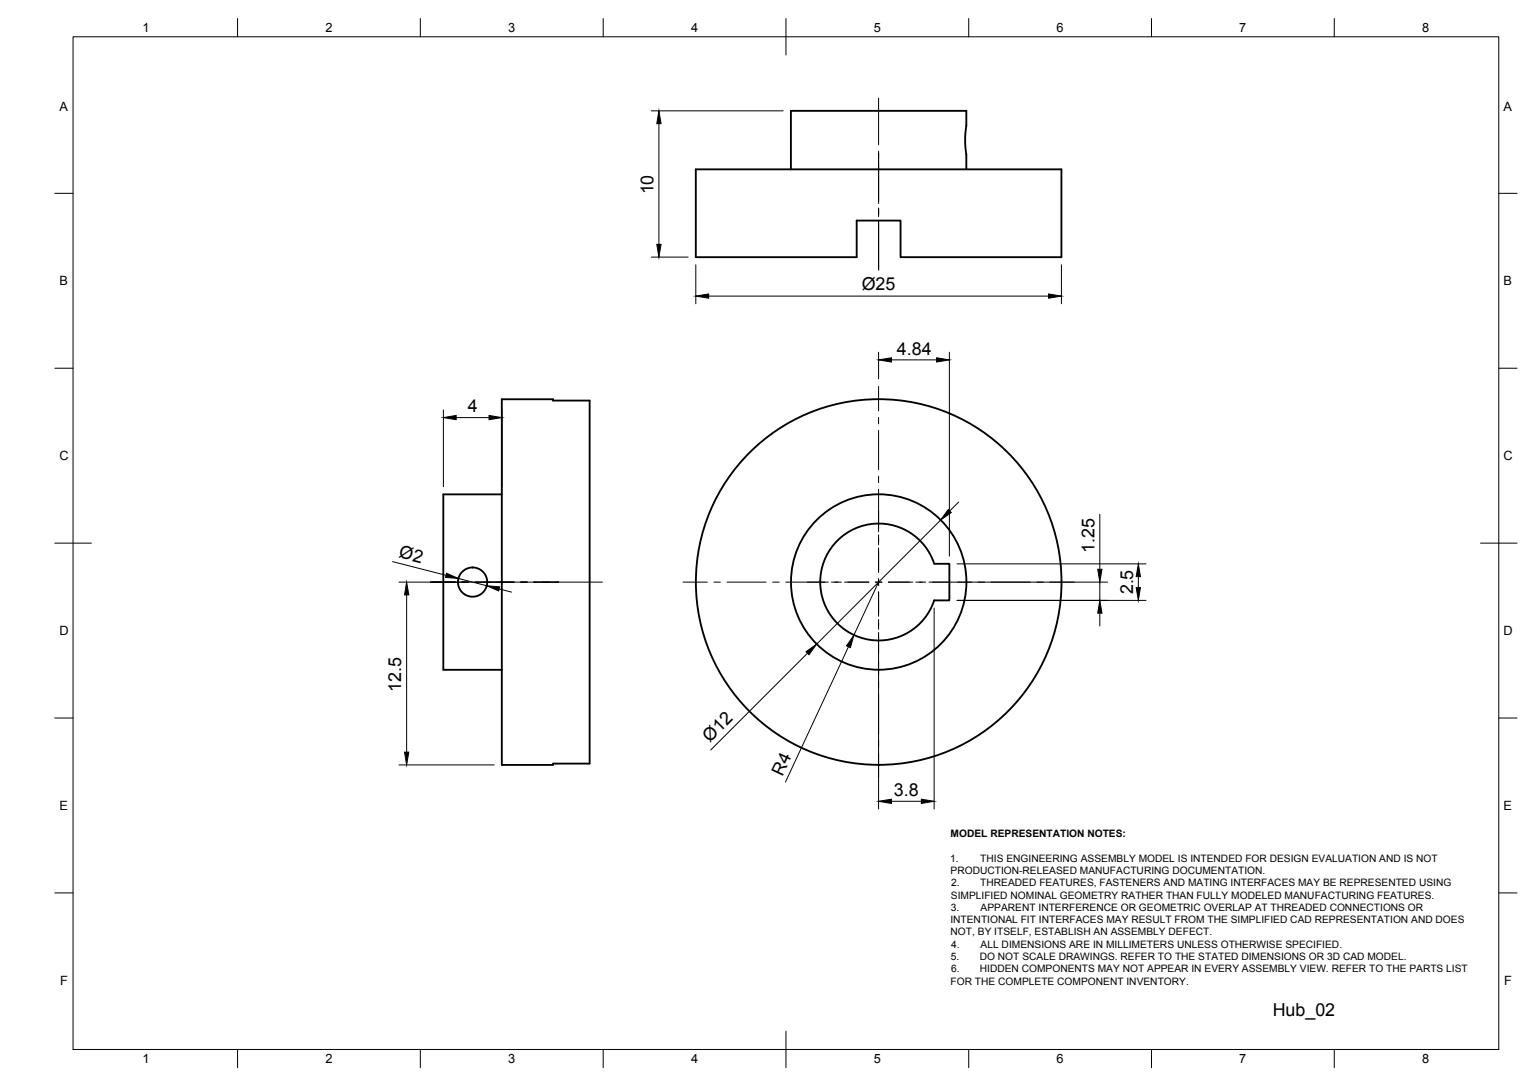
ISO-10303-21;
HEADER;
/* Generated by software containing ST-Developer
 * from STEP Tools, Inc. (www.steptools.com) 
 */

FILE_DESCRIPTION(
/* description */ (''),
/* implementation_level */ '2;1');

FILE_NAME(
/* name */ 'Hub_02.step',
/* time_stamp */ '2026-10-05T22:24:12-07:00',
/* author */ (''),
/* organization */ (''),
/* preprocessor_version */ 'ST-DEVELOPER v20.2',
/* originating_system */ 'Autodesk Translation Framework v15.15.0.0',
/* authorisation */ '');

FILE_SCHEMA (('AUTOMOTIVE_DESIGN { 1 0 10303 214 3 1 1 }'));
ENDSEC;

DATA;
#10=MECHANICAL_DESIGN_GEOMETRIC_PRESENTATION_REPRESENTATION('',(#55),#2116);
#41=SHAPE_REPRESENTATION_RELATIONSHIP('SRR','None',#2147,#48);
#48=ADVANCED_BREP_SHAPE_REPRESENTATION('',(#62),#2111);
#55=STYLED_ITEM('',(#2191),#62);
#62=MANIFOLD_SOLID_BREP('Body1',#1149);
#71=FACE_BOUND('',#230,.T.);
#72=FACE_BOUND('',#234,.T.);
#73=FACE_BOUND('',#237,.T.);
#74=FACE_BOUND('',#239,.T.);
#96=PLANE('',#1285);
#97=PLANE('',#1286);
#98=PLANE('',#1287);
#99=PLANE('',#1288);
#100=PLANE('',#1295);
#101=PLANE('',#1297);
#102=PLANE('',#1298);
#103=PLANE('',#1299);
#104=PLANE('',#1303);
#105=PLANE('',#1305);
#106=PLANE('',#1308);
#157=FACE_OUTER_BOUND('',#228,.T.);
#158=FACE_OUTER_BOUND('',#229,.T.);
#159=FACE_OUTER_BOUND('',#231,.T.);
#160=FACE_OUTER_BOUND('',#232,.T.);
#161=FACE_OUTER_BOUND('',#233,.T.);
#162=FACE_OUTER_BOUND('',#235,.T.);
#163=FACE_OUTER_BOUND('',#236,.T.);
#164=FACE_OUTER_BOUND('',#238,.T.);
#165=FACE_OUTER_BOUND('',#240,.T.);
#166=FACE_OUTER_BOUND('',#241,.T.);
#167=FACE_OUTER_BOUND('',#242,.T.);
#168=FACE_OUTER_BOUND('',#243,.T.);
#169=FACE_OUTER_BOUND('',#244,.T.);
#170=FACE_OUTER_BOUND('',#245,.T.);
#171=FACE_OUTER_BOUND('',#246,.T.);
#228=EDGE_LOOP('',(#893,#894,#895,#896,#897));
#229=EDGE_LOOP('',(#898,#899,#900,#901));
#230=EDGE_LOOP('',(#902));
#231=EDGE_LOOP('',(#903,#904,#905,#906));
#232=EDGE_LOOP('',(#907,#908,#909,#910));
#233=EDGE_LOOP('',(#911));
#234=EDGE_LOOP('',(#912,#913,#914,#915));
#235=EDGE_LOOP('',(#916,#917,#918,#919));
#236=EDGE_LOOP('',(#920,#921,#922,#923));
#237=EDGE_LOOP('',(#924,#925));
#238=EDGE_LOOP('',(#926));
#239=EDGE_LOOP('',(#927));
#240=EDGE_LOOP('',(#928,#929,#930,#931));
#241=EDGE_LOOP('',(#932,#933,#934,#935));
#242=EDGE_LOOP('',(#936,#937,#938,#939,#940));
#243=EDGE_LOOP('',(#941,#942));
#244=EDGE_LOOP('',(#943,#944));
#245=EDGE_LOOP('',(#945,#946,#947,#948,#949,#950,#951,#952,#953,#954,#955,
#956));
#246=EDGE_LOOP('',(#957,#958,#959,#960));
#274=B_SPLINE_CURVE_WITH_KNOTS('',3,(#1872,#1873,#1874,#1875,#1876,#1877,
#1878,#1879,#1880,#1881,#1882,#1883,#1884,#1885,#1886,#1887,#1888,#1889),
 .UNSPECIFIED.,.F.,.F.,(4,2,2,2,2,2,2,2,4),(0.,0.0377449625945587,0.0754899251891175,
0.113233879657538,0.150977834125959,0.18872178859438,0.226465743062801,
0.264210705657359,0.301955668251918),.UNSPECIFIED.);
#275=B_SPLINE_CURVE_WITH_KNOTS('',3,(#1890,#1891,#1892,#1893,#1894,#1895,
#1896,#1897,#1898,#1899,#1900,#1901,#1902,#1903,#1904,#1905,#1906,#1907),
 .UNSPECIFIED.,.F.,.F.,(4,2,2,2,2,2,2,2,4),(0.301955668251918,0.339700630846477,
0.377445593441036,0.415189547909457,0.452933502377877,0.490677456846298,
0.528421411314719,0.566166373909278,0.603911336503836),.UNSPECIFIED.);
#314=LINE('',#1870,#419);
#315=LINE('',#1911,#420);
#316=LINE('',#1913,#421);
#317=LINE('',#1915,#422);
#318=LINE('',#1916,#423);
#319=LINE('',#1919,#424);
#320=LINE('',#1921,#425);
#321=LINE('',#1922,#426);
#322=LINE('',#1925,#427);
#323=LINE('',#1927,#428);
#324=LINE('',#1928,#429);
#325=LINE('',#1937,#430);
#326=LINE('',#1945,#431);
#327=LINE('',#1947,#432);
#328=LINE('',#1949,#433);
#329=LINE('',#1950,#434);
#330=LINE('',#1954,#435);
#331=LINE('',#1956,#436);
#332=LINE('',#1958,#437);
#333=LINE('',#1959,#438);
#334=LINE('',#1970,#439);
#419=VECTOR('',#1498,0.999999999999999);
#420=VECTOR('',#1501,10.);
#421=VECTOR('',#1502,10.);
#422=VECTOR('',#1503,10.);
#423=VECTOR('',#1504,10.);
#424=VECTOR('',#1507,10.);
#425=VECTOR('',#1508,10.);
#426=VECTOR('',#1509,10.);
#427=VECTOR('',#1512,10.);
#428=VECTOR('',#1513,10.);
#429=VECTOR('',#1514,10.);
#430=VECTOR('',#1527,6.);
#431=VECTOR('',#1536,10.);
#432=VECTOR('',#1537,10.);
#433=VECTOR('',#1538,10.);
#434=VECTOR('',#1539,10.);
#435=VECTOR('',#1542,10.);
#436=VECTOR('',#1543,10.);
#437=VECTOR('',#1544,10.);
#438=VECTOR('',#1545,10.);
#439=VECTOR('',#1564,12.5);
#507=CIRCLE('',#1284,0.999999999999999);
#508=CIRCLE('',#1289,6.);
#509=CIRCLE('',#1290,4.);
#510=CIRCLE('',#1292,4.);
#511=CIRCLE('',#1294,6.);
#512=CIRCLE('',#1296,12.5);
#513=CIRCLE('',#1300,12.5);
#514=CIRCLE('',#1301,12.5);
#515=CIRCLE('',#1302,12.5);
#516=CIRCLE('',#1304,12.5);
#517=CIRCLE('',#1306,12.5);
#566=VERTEX_POINT('',#1867);
#567=VERTEX_POINT('',#1869);
#568=VERTEX_POINT('',#1871);
#569=VERTEX_POINT('',#1909);
#570=VERTEX_POINT('',#1910);
#571=VERTEX_POINT('',#1912);
#572=VERTEX_POINT('',#1914);
#573=VERTEX_POINT('',#1918);
#574=VERTEX_POINT('',#1920);
#575=VERTEX_POINT('',#1924);
#576=VERTEX_POINT('',#1926);
#577=VERTEX_POINT('',#1930);
#578=VERTEX_POINT('',#1936);
#579=VERTEX_POINT('',#1940);
#580=VERTEX_POINT('',#1943);
#581=VERTEX_POINT('',#1944);
#582=VERTEX_POINT('',#1946);
#583=VERTEX_POINT('',#1948);
#584=VERTEX_POINT('',#1952);
#585=VERTEX_POINT('',#1953);
#586=VERTEX_POINT('',#1955);
#587=VERTEX_POINT('',#1957);
#588=VERTEX_POINT('',#1962);
#685=EDGE_CURVE('',#566,#566,#507,.T.);
#686=EDGE_CURVE('',#566,#567,#314,.T.);
#687=EDGE_CURVE('',#568,#567,#274,.T.);
#688=EDGE_CURVE('',#567,#568,#275,.T.);
#689=EDGE_CURVE('',#569,#570,#315,.T.);
#690=EDGE_CURVE('',#571,#569,#316,.T.);
#691=EDGE_CURVE('',#572,#571,#317,.T.);
#692=EDGE_CURVE('',#572,#570,#318,.T.);
#693=EDGE_CURVE('',#570,#573,#319,.T.);
#694=EDGE_CURVE('',#572,#574,#320,.T.);
#695=EDGE_CURVE('',#573,#574,#321,.T.);
#696=EDGE_CURVE('',#575,#569,#322,.T.);
#697=EDGE_CURVE('',#576,#575,#323,.T.);
#698=EDGE_CURVE('',#571,#576,#324,.T.);
#699=EDGE_CURVE('',#577,#577,#508,.T.);
#700=EDGE_CURVE('',#573,#575,#509,.T.);
#701=EDGE_CURVE('',#576,#574,#510,.T.);
#702=EDGE_CURVE('',#577,#578,#325,.T.);
#703=EDGE_CURVE('',#578,#578,#511,.T.);
#704=EDGE_CURVE('',#579,#579,#512,.T.);
#705=EDGE_CURVE('',#580,#581,#326,.T.);
#706=EDGE_CURVE('',#582,#580,#327,.T.);
#707=EDGE_CURVE('',#582,#583,#328,.T.);
#708=EDGE_CURVE('',#581,#583,#329,.T.);
#709=EDGE_CURVE('',#584,#585,#330,.T.);
#710=EDGE_CURVE('',#586,#584,#331,.T.);
#711=EDGE_CURVE('',#586,#587,#332,.T.);
#712=EDGE_CURVE('',#585,#587,#333,.T.);
#713=EDGE_CURVE('',#583,#586,#513,.T.);
#714=EDGE_CURVE('',#588,#582,#514,.T.);
#715=EDGE_CURVE('',#587,#588,#515,.T.);
#716=EDGE_CURVE('',#584,#585,#516,.T.);
#717=EDGE_CURVE('',#580,#581,#517,.T.);
#718=EDGE_CURVE('',#579,#588,#334,.T.);
#893=ORIENTED_EDGE('',*,*,#685,.F.);
#894=ORIENTED_EDGE('',*,*,#686,.T.);
#895=ORIENTED_EDGE('',*,*,#687,.F.);
#896=ORIENTED_EDGE('',*,*,#688,.F.);
#897=ORIENTED_EDGE('',*,*,#686,.F.);
#898=ORIENTED_EDGE('',*,*,#689,.F.);
#899=ORIENTED_EDGE('',*,*,#690,.F.);
#900=ORIENTED_EDGE('',*,*,#691,.F.);
#901=ORIENTED_EDGE('',*,*,#692,.T.);
#902=ORIENTED_EDGE('',*,*,#685,.T.);
#903=ORIENTED_EDGE('',*,*,#693,.F.);
#904=ORIENTED_EDGE('',*,*,#692,.F.);
#905=ORIENTED_EDGE('',*,*,#694,.T.);
#906=ORIENTED_EDGE('',*,*,#695,.F.);
#907=ORIENTED_EDGE('',*,*,#696,.F.);
#908=ORIENTED_EDGE('',*,*,#697,.F.);
#909=ORIENTED_EDGE('',*,*,#698,.F.);
#910=ORIENTED_EDGE('',*,*,#690,.T.);
#911=ORIENTED_EDGE('',*,*,#699,.T.);
#912=ORIENTED_EDGE('',*,*,#696,.T.);
#913=ORIENTED_EDGE('',*,*,#689,.T.);
#914=ORIENTED_EDGE('',*,*,#693,.T.);
#915=ORIENTED_EDGE('',*,*,#700,.T.);
#916=ORIENTED_EDGE('',*,*,#697,.T.);
#917=ORIENTED_EDGE('',*,*,#700,.F.);
#918=ORIENTED_EDGE('',*,*,#695,.T.);
#919=ORIENTED_EDGE('',*,*,#701,.F.);
#920=ORIENTED_EDGE('',*,*,#699,.F.);
#921=ORIENTED_EDGE('',*,*,#702,.T.);
#922=ORIENTED_EDGE('',*,*,#703,.F.);
#923=ORIENTED_EDGE('',*,*,#702,.F.);
#924=ORIENTED_EDGE('',*,*,#687,.T.);
#925=ORIENTED_EDGE('',*,*,#688,.T.);
#926=ORIENTED_EDGE('',*,*,#704,.T.);
#927=ORIENTED_EDGE('',*,*,#703,.T.);
#928=ORIENTED_EDGE('',*,*,#705,.F.);
#929=ORIENTED_EDGE('',*,*,#706,.F.);
#930=ORIENTED_EDGE('',*,*,#707,.T.);
#931=ORIENTED_EDGE('',*,*,#708,.F.);
#932=ORIENTED_EDGE('',*,*,#709,.F.);
#933=ORIENTED_EDGE('',*,*,#710,.F.);
#934=ORIENTED_EDGE('',*,*,#711,.T.);
#935=ORIENTED_EDGE('',*,*,#712,.F.);
#936=ORIENTED_EDGE('',*,*,#713,.F.);
#937=ORIENTED_EDGE('',*,*,#707,.F.);
#938=ORIENTED_EDGE('',*,*,#714,.F.);
#939=ORIENTED_EDGE('',*,*,#715,.F.);
#940=ORIENTED_EDGE('',*,*,#711,.F.);
#941=ORIENTED_EDGE('',*,*,#709,.T.);
#942=ORIENTED_EDGE('',*,*,#716,.F.);
#943=ORIENTED_EDGE('',*,*,#705,.T.);
#944=ORIENTED_EDGE('',*,*,#717,.F.);
#945=ORIENTED_EDGE('',*,*,#704,.F.);
#946=ORIENTED_EDGE('',*,*,#718,.T.);
#947=ORIENTED_EDGE('',*,*,#714,.T.);
#948=ORIENTED_EDGE('',*,*,#706,.T.);
#949=ORIENTED_EDGE('',*,*,#717,.T.);
#950=ORIENTED_EDGE('',*,*,#708,.T.);
#951=ORIENTED_EDGE('',*,*,#713,.T.);
#952=ORIENTED_EDGE('',*,*,#710,.T.);
#953=ORIENTED_EDGE('',*,*,#716,.T.);
#954=ORIENTED_EDGE('',*,*,#712,.T.);
#955=ORIENTED_EDGE('',*,*,#715,.T.);
#956=ORIENTED_EDGE('',*,*,#718,.F.);
#957=ORIENTED_EDGE('',*,*,#701,.T.);
#958=ORIENTED_EDGE('',*,*,#694,.F.);
#959=ORIENTED_EDGE('',*,*,#691,.T.);
#960=ORIENTED_EDGE('',*,*,#698,.T.);
#1074=CYLINDRICAL_SURFACE('',#1283,0.999999999999999);
#1075=CYLINDRICAL_SURFACE('',#1291,4.);
#1076=CYLINDRICAL_SURFACE('',#1293,6.);
#1077=CYLINDRICAL_SURFACE('',#1307,12.5);
#1106=ADVANCED_FACE('',(#157),#1074,.F.);
#1107=ADVANCED_FACE('',(#158,#71),#96,.T.);
#1108=ADVANCED_FACE('',(#159),#97,.T.);
#1109=ADVANCED_FACE('',(#160),#98,.T.);
#1110=ADVANCED_FACE('',(#161,#72),#99,.T.);
#1111=ADVANCED_FACE('',(#162),#1075,.F.);
#1112=ADVANCED_FACE('',(#163,#73),#1076,.T.);
#1113=ADVANCED_FACE('',(#164,#74),#100,.T.);
#1114=ADVANCED_FACE('',(#165),#101,.F.);
#1115=ADVANCED_FACE('',(#166),#102,.F.);
#1116=ADVANCED_FACE('',(#167),#103,.F.);
#1117=ADVANCED_FACE('',(#168),#104,.F.);
#1118=ADVANCED_FACE('',(#169),#105,.F.);
#1119=ADVANCED_FACE('',(#170),#1077,.T.);
#1120=ADVANCED_FACE('',(#171),#106,.T.);
#1149=CLOSED_SHELL('',(#1106,#1107,#1108,#1109,#1110,#1111,#1112,#1113,
#1114,#1115,#1116,#1117,#1118,#1119,#1120));
#1282=AXIS2_PLACEMENT_3D('',#1865,#1492,#1493);
#1283=AXIS2_PLACEMENT_3D('',#1866,#1494,#1495);
#1284=AXIS2_PLACEMENT_3D('',#1868,#1496,#1497);
#1285=AXIS2_PLACEMENT_3D('',#1908,#1499,#1500);
#1286=AXIS2_PLACEMENT_3D('',#1917,#1505,#1506);
#1287=AXIS2_PLACEMENT_3D('',#1923,#1510,#1511);
#1288=AXIS2_PLACEMENT_3D('',#1929,#1515,#1516);
#1289=AXIS2_PLACEMENT_3D('',#1931,#1517,#1518);
#1290=AXIS2_PLACEMENT_3D('',#1932,#1519,#1520);
#1291=AXIS2_PLACEMENT_3D('',#1933,#1521,#1522);
#1292=AXIS2_PLACEMENT_3D('',#1934,#1523,#1524);
#1293=AXIS2_PLACEMENT_3D('',#1935,#1525,#1526);
#1294=AXIS2_PLACEMENT_3D('',#1938,#1528,#1529);
#1295=AXIS2_PLACEMENT_3D('',#1939,#1530,#1531);
#1296=AXIS2_PLACEMENT_3D('',#1941,#1532,#1533);
#1297=AXIS2_PLACEMENT_3D('',#1942,#1534,#1535);
#1298=AXIS2_PLACEMENT_3D('',#1951,#1540,#1541);
#1299=AXIS2_PLACEMENT_3D('',#1960,#1546,#1547);
#1300=AXIS2_PLACEMENT_3D('',#1961,#1548,#1549);
#1301=AXIS2_PLACEMENT_3D('',#1963,#1550,#1551);
#1302=AXIS2_PLACEMENT_3D('',#1964,#1552,#1553);
#1303=AXIS2_PLACEMENT_3D('',#1965,#1554,#1555);
#1304=AXIS2_PLACEMENT_3D('',#1966,#1556,#1557);
#1305=AXIS2_PLACEMENT_3D('',#1967,#1558,#1559);
#1306=AXIS2_PLACEMENT_3D('',#1968,#1560,#1561);
#1307=AXIS2_PLACEMENT_3D('',#1969,#1562,#1563);
#1308=AXIS2_PLACEMENT_3D('',#1971,#1565,#1566);
#1492=DIRECTION('axis',(0.,0.,1.));
#1493=DIRECTION('refdir',(1.,0.,0.));
#1494=DIRECTION('center_axis',(0.,0.,1.));
#1495=DIRECTION('ref_axis',(1.,0.,0.));
#1496=DIRECTION('center_axis',(0.,0.,1.));
#1497=DIRECTION('ref_axis',(1.,0.,0.));
#1498=DIRECTION('',(0.,0.,1.));
#1499=DIRECTION('center_axis',(0.,0.,-1.));
#1500=DIRECTION('ref_axis',(-1.,0.,0.));
#1501=DIRECTION('',(-1.,0.,0.));
#1502=DIRECTION('',(0.,1.,0.));
#1503=DIRECTION('',(1.,0.,0.));
#1504=DIRECTION('',(0.,1.,0.));
#1505=DIRECTION('center_axis',(1.,0.,0.));
#1506=DIRECTION('ref_axis',(0.,0.,-1.));
#1507=DIRECTION('',(0.,0.,-1.));
#1508=DIRECTION('',(0.,0.,-1.));
#1509=DIRECTION('',(0.,-1.,0.));
#1510=DIRECTION('center_axis',(-1.,0.,0.));
#1511=DIRECTION('ref_axis',(0.,0.,1.));
#1512=DIRECTION('',(0.,0.,1.));
#1513=DIRECTION('',(0.,1.,0.));
#1514=DIRECTION('',(0.,0.,-1.));
#1515=DIRECTION('center_axis',(0.,1.,0.));
#1516=DIRECTION('ref_axis',(-1.,0.,0.));
#1517=DIRECTION('center_axis',(0.,1.,0.));
#1518=DIRECTION('ref_axis',(-1.,0.,0.));
#1519=DIRECTION('center_axis',(0.,-1.,0.));
#1520=DIRECTION('ref_axis',(-1.,0.,0.));
#1521=DIRECTION('center_axis',(0.,1.,0.));
#1522=DIRECTION('ref_axis',(1.83697019872103E-16,0.,-1.));
#1523=DIRECTION('center_axis',(0.,1.,0.));
#1524=DIRECTION('ref_axis',(-1.,0.,0.));
#1525=DIRECTION('center_axis',(0.,1.,0.));
#1526=DIRECTION('ref_axis',(-1.,0.,0.));
#1527=DIRECTION('',(0.,-1.,0.));
#1528=DIRECTION('center_axis',(0.,-1.,0.));
#1529=DIRECTION('ref_axis',(-1.,0.,0.));
#1530=DIRECTION('center_axis',(0.,1.,0.));
#1531=DIRECTION('ref_axis',(-1.,0.,0.));
#1532=DIRECTION('center_axis',(0.,1.,0.));
#1533=DIRECTION('ref_axis',(-1.,0.,0.));
#1534=DIRECTION('center_axis',(0.,0.,-1.));
#1535=DIRECTION('ref_axis',(-1.,0.,0.));
#1536=DIRECTION('',(-1.,0.,0.));
#1537=DIRECTION('',(0.,-1.,0.));
#1538=DIRECTION('',(-1.,0.,0.));
#1539=DIRECTION('',(0.,1.,0.));
#1540=DIRECTION('center_axis',(0.,0.,1.));
#1541=DIRECTION('ref_axis',(1.,0.,0.));
#1542=DIRECTION('',(1.,0.,0.));
#1543=DIRECTION('',(0.,-1.,0.));
#1544=DIRECTION('',(1.,0.,0.));
#1545=DIRECTION('',(0.,1.,0.));
#1546=DIRECTION('center_axis',(0.,1.,0.));
#1547=DIRECTION('ref_axis',(-1.,0.,0.));
#1548=DIRECTION('center_axis',(0.,1.,0.));
#1549=DIRECTION('ref_axis',(-1.,0.,0.));
#1550=DIRECTION('center_axis',(0.,1.,0.));
#1551=DIRECTION('ref_axis',(-1.,0.,0.));
#1552=DIRECTION('center_axis',(0.,1.,0.));
#1553=DIRECTION('ref_axis',(-1.,0.,0.));
#1554=DIRECTION('center_axis',(0.,1.,0.));
#1555=DIRECTION('ref_axis',(-1.,0.,0.));
#1556=DIRECTION('center_axis',(0.,1.,0.));
#1557=DIRECTION('ref_axis',(-1.,0.,0.));
#1558=DIRECTION('center_axis',(0.,1.,0.));
#1559=DIRECTION('ref_axis',(-1.,0.,0.));
#1560=DIRECTION('center_axis',(0.,1.,0.));
#1561=DIRECTION('ref_axis',(-1.,0.,0.));
#1562=DIRECTION('center_axis',(0.,1.,0.));
#1563=DIRECTION('ref_axis',(-1.,0.,0.));
#1564=DIRECTION('',(0.,-1.,0.));
#1565=DIRECTION('center_axis',(0.,1.,0.));
#1566=DIRECTION('ref_axis',(-1.,0.,0.));
#1865=CARTESIAN_POINT('',(0.,0.,0.));
#1866=CARTESIAN_POINT('Origin',(2.,12.,2.));
#1867=CARTESIAN_POINT('',(1.,12.,6.84122918275927));
#1868=CARTESIAN_POINT('Origin',(2.,12.,6.84122918275927));
#1869=CARTESIAN_POINT('',(1.,12.,7.91607978309962));
#1870=CARTESIAN_POINT('',(1.,12.,2.));
#1871=CARTESIAN_POINT('',(3.,12.,7.91607978309962));
#1872=CARTESIAN_POINT('Ctrl Pts',(3.,12.,7.91607978309962));
#1873=CARTESIAN_POINT('Ctrl Pts',(3.,11.8741834580181,7.91607978309962));
#1874=CARTESIAN_POINT('Ctrl Pts',(2.97480737102551,11.7401445190311,7.92050853647266));
#1875=CARTESIAN_POINT('Ctrl Pts',(2.87268154620344,11.493836747049,7.93642128117897));
#1876=CARTESIAN_POINT('Ctrl Pts',(2.79576089648453,11.3815473341114,7.94766633611059));
#1877=CARTESIAN_POINT('Ctrl Pts',(2.61845503374177,11.2042414713687,7.96870867068992));
#1878=CARTESIAN_POINT('Ctrl Pts',(2.50616460424207,11.1273189643764,7.97988517961729));
#1879=CARTESIAN_POINT('Ctrl Pts',(2.25985334006496,11.0251917910001,7.99564055034545));
#1880=CARTESIAN_POINT('Ctrl Pts',(2.1258131815614,11.,8.));
#1881=CARTESIAN_POINT('Ctrl Pts',(1.8741868184386,11.,8.));
#1882=CARTESIAN_POINT('Ctrl Pts',(1.74014665993504,11.0251917910001,7.99564055034545));
#1883=CARTESIAN_POINT('Ctrl Pts',(1.49383539575793,11.1273189643764,7.97988517961729));
#1884=CARTESIAN_POINT('Ctrl Pts',(1.38154496625823,11.2042414713687,7.96870867068992));
#1885=CARTESIAN_POINT('Ctrl Pts',(1.20423910351547,11.3815473341114,7.94766633611059));
#1886=CARTESIAN_POINT('Ctrl Pts',(1.12731845379656,11.493836747049,7.93642128117897));
#1887=CARTESIAN_POINT('Ctrl Pts',(1.02519262897449,11.7401445190311,7.92050853647266));
#1888=CARTESIAN_POINT('Ctrl Pts',(1.,11.8741834580181,7.91607978309962));
#1889=CARTESIAN_POINT('Ctrl Pts',(1.,12.,7.91607978309962));
#1890=CARTESIAN_POINT('Ctrl Pts',(1.,12.,7.91607978309962));
#1891=CARTESIAN_POINT('Ctrl Pts',(1.,12.1258165419819,7.91607978309962));
#1892=CARTESIAN_POINT('Ctrl Pts',(1.02519262897449,12.2598554809689,7.92050853647266));
#1893=CARTESIAN_POINT('Ctrl Pts',(1.12731845379656,12.506163252951,7.93642128117897));
#1894=CARTESIAN_POINT('Ctrl Pts',(1.20423910351547,12.6184526658886,7.94766633611059));
#1895=CARTESIAN_POINT('Ctrl Pts',(1.38154496625823,12.7957585286313,7.96870867068992));
#1896=CARTESIAN_POINT('Ctrl Pts',(1.49383539575793,12.8726810356236,7.97988517961729));
#1897=CARTESIAN_POINT('Ctrl Pts',(1.74014665993504,12.9748082089999,7.99564055034545));
#1898=CARTESIAN_POINT('Ctrl Pts',(1.8741868184386,13.,8.));
#1899=CARTESIAN_POINT('Ctrl Pts',(2.1258131815614,13.,8.));
#1900=CARTESIAN_POINT('Ctrl Pts',(2.25985334006496,12.9748082089999,7.99564055034545));
#1901=CARTESIAN_POINT('Ctrl Pts',(2.50616460424207,12.8726810356236,7.97988517961729));
#1902=CARTESIAN_POINT('Ctrl Pts',(2.61845503374177,12.7957585286313,7.96870867068992));
#1903=CARTESIAN_POINT('Ctrl Pts',(2.79576089648453,12.6184526658886,7.94766633611059));
#1904=CARTESIAN_POINT('Ctrl Pts',(2.87268154620344,12.506163252951,7.93642128117897));
#1905=CARTESIAN_POINT('Ctrl Pts',(2.97480737102551,12.2598554809689,7.92050853647266));
#1906=CARTESIAN_POINT('Ctrl Pts',(3.,12.1258165419819,7.91607978309962));
#1907=CARTESIAN_POINT('Ctrl Pts',(3.,12.,7.91607978309962));
#1908=CARTESIAN_POINT('Origin',(3.25,10.,6.84122918275927));
#1909=CARTESIAN_POINT('',(3.25,14.,6.84122918275927));
#1910=CARTESIAN_POINT('',(0.75,14.,6.84122918275927));
#1911=CARTESIAN_POINT('',(2.625,14.,6.84122918275927));
#1912=CARTESIAN_POINT('',(3.25,10.,6.84122918275927));
#1913=CARTESIAN_POINT('',(3.25,10.,6.84122918275927));
#1914=CARTESIAN_POINT('',(0.75,10.,6.84122918275927));
#1915=CARTESIAN_POINT('',(0.75,10.,6.84122918275927));
#1916=CARTESIAN_POINT('',(0.75,10.,6.84122918275927));
#1917=CARTESIAN_POINT('Origin',(0.75,10.,6.84122918275927));
#1918=CARTESIAN_POINT('',(0.75,14.,5.79967103839267));
#1919=CARTESIAN_POINT('',(0.75,14.,4.42061459137964));
#1920=CARTESIAN_POINT('',(0.75,10.,5.79967103839267));
#1921=CARTESIAN_POINT('',(0.75,10.,5.79967103839267));
#1922=CARTESIAN_POINT('',(0.75,10.,5.79967103839267));
#1923=CARTESIAN_POINT('Origin',(3.25,10.,5.29967103839267));
#1924=CARTESIAN_POINT('',(3.25,14.,5.79967103839267));
#1925=CARTESIAN_POINT('',(3.25,14.,3.64983551919633));
#1926=CARTESIAN_POINT('',(3.25,10.,5.79967103839267));
#1927=CARTESIAN_POINT('',(3.25,10.,5.79967103839267));
#1928=CARTESIAN_POINT('',(3.25,10.,8.32461990770089));
#1929=CARTESIAN_POINT('Origin',(2.,14.,2.));
#1930=CARTESIAN_POINT('',(8.,14.,2.));
#1931=CARTESIAN_POINT('Origin',(2.,14.,2.));
#1932=CARTESIAN_POINT('Origin',(2.,14.,2.));
#1933=CARTESIAN_POINT('Origin',(2.,10.,2.));
#1934=CARTESIAN_POINT('Origin',(2.,10.,2.));
#1935=CARTESIAN_POINT('Origin',(2.,10.,2.));
#1936=CARTESIAN_POINT('',(8.,10.,2.));
#1937=CARTESIAN_POINT('',(8.,10.,2.));
#1938=CARTESIAN_POINT('Origin',(2.,10.,2.));
#1939=CARTESIAN_POINT('Origin',(2.,10.,2.));
#1940=CARTESIAN_POINT('',(14.5,10.,2.));
#1941=CARTESIAN_POINT('Origin',(2.,10.,2.));
#1942=CARTESIAN_POINT('Origin',(14.4096736459909,4.,0.499999999999999));
#1943=CARTESIAN_POINT('',(14.4096736459909,4.,0.499999999999999));
#1944=CARTESIAN_POINT('',(-10.4096736459909,4.,0.499999999999999));
#1945=CARTESIAN_POINT('',(8.20483682299543,4.,0.499999999999999));
#1946=CARTESIAN_POINT('',(14.4096736459909,6.5,0.499999999999999));
#1947=CARTESIAN_POINT('',(14.4096736459909,4.,0.499999999999999));
#1948=CARTESIAN_POINT('',(-10.4096736459909,6.5,0.499999999999999));
#1949=CARTESIAN_POINT('',(-16.9791024697249,6.5,0.499999999999999));
#1950=CARTESIAN_POINT('',(-10.4096736459909,4.,0.499999999999999));
#1951=CARTESIAN_POINT('Origin',(-10.4096736459909,4.,3.5));
#1952=CARTESIAN_POINT('',(-10.4096736459909,4.,3.5));
#1953=CARTESIAN_POINT('',(14.4096736459909,4.,3.5));
#1954=CARTESIAN_POINT('',(-4.20483682299543,4.,3.5));
#1955=CARTESIAN_POINT('',(-10.4096736459909,6.5,3.5));
#1956=CARTESIAN_POINT('',(-10.4096736459909,4.,3.5));
#1957=CARTESIAN_POINT('',(14.4096736459909,6.5,3.5));
#1958=CARTESIAN_POINT('',(20.9791024697249,6.5,3.5));
#1959=CARTESIAN_POINT('',(14.4096736459909,4.,3.5));
#1960=CARTESIAN_POINT('Origin',(2.,6.5,2.));
#1961=CARTESIAN_POINT('Origin',(2.,6.5,2.));
#1962=CARTESIAN_POINT('',(14.5,6.5,2.));
#1963=CARTESIAN_POINT('Origin',(2.,6.5,2.));
#1964=CARTESIAN_POINT('Origin',(2.,6.5,2.));
#1965=CARTESIAN_POINT('Origin',(2.,4.,2.));
#1966=CARTESIAN_POINT('Origin',(2.,4.,2.));
#1967=CARTESIAN_POINT('Origin',(2.,4.,2.));
#1968=CARTESIAN_POINT('Origin',(2.,4.,2.));
#1969=CARTESIAN_POINT('Origin',(2.,4.,2.));
#1970=CARTESIAN_POINT('',(14.5,4.,2.));
#1971=CARTESIAN_POINT('Origin',(2.,10.,2.));
#2102=UNCERTAINTY_MEASURE_WITH_UNIT(LENGTH_MEASURE(0.01),#2117,
'DISTANCE_ACCURACY_VALUE',
'Maximum model space distance between geometric entities at asserted c
onnectivities');
#2107=UNCERTAINTY_MEASURE_WITH_UNIT(LENGTH_MEASURE(0.01),#2117,
'DISTANCE_ACCURACY_VALUE',
'Maximum model space distance between geometric entities at asserted c
onnectivities');
#2111=(
GEOMETRIC_REPRESENTATION_CONTEXT(3)
GLOBAL_UNCERTAINTY_ASSIGNED_CONTEXT((#2102))
GLOBAL_UNIT_ASSIGNED_CONTEXT((#2117,#2119,#2120))
REPRESENTATION_CONTEXT('','3D')
);
#2116=(
GEOMETRIC_REPRESENTATION_CONTEXT(3)
GLOBAL_UNCERTAINTY_ASSIGNED_CONTEXT((#2107))
GLOBAL_UNIT_ASSIGNED_CONTEXT((#2117,#2119,#2120))
REPRESENTATION_CONTEXT('','3D')
);
#2117=(
LENGTH_UNIT()
NAMED_UNIT(*)
SI_UNIT(.MILLI.,.METRE.)
);
#2119=(
NAMED_UNIT(*)
PLANE_ANGLE_UNIT()
SI_UNIT($,.RADIAN.)
);
#2120=(
NAMED_UNIT(*)
SI_UNIT($,.STERADIAN.)
SOLID_ANGLE_UNIT()
);
#2124=SHAPE_DEFINITION_REPRESENTATION(#2132,#2147);
#2132=PRODUCT_DEFINITION_SHAPE('',$,#2156);
#2147=SHAPE_REPRESENTATION('',(#1282),#2111);
#2152=PRODUCT_DEFINITION_CONTEXT('part definition',#2178,'design');
#2156=PRODUCT_DEFINITION('Hub_02','Hub_02',#2164,#2152);
#2164=PRODUCT_DEFINITION_FORMATION('',$,#2183);
#2178=APPLICATION_CONTEXT(
'Core Data for Automotive Mechanical Design Process');
#2179=PRODUCT_CONTEXT('part definition',#2178,'mechanical');
#2183=PRODUCT('Hub_02','Hub_02',$,(#2179));
#2191=PRESENTATION_STYLE_ASSIGNMENT((#2196));
#2196=SURFACE_STYLE_USAGE(.BOTH.,#2201);
#2201=SURFACE_SIDE_STYLE('',(#2206));
#2206=SURFACE_STYLE_FILL_AREA(#2211);
#2211=FILL_AREA_STYLE('Opaque(224,224,112)',(#2216));
#2216=FILL_AREA_STYLE_COLOUR('Opaque(224,224,112)',#2221);
#2221=COLOUR_RGB('Opaque(224,224,112)', 0.31764706, 0.68627451, 0.89019608);
ENDSEC;
END-ISO-10303-21;
